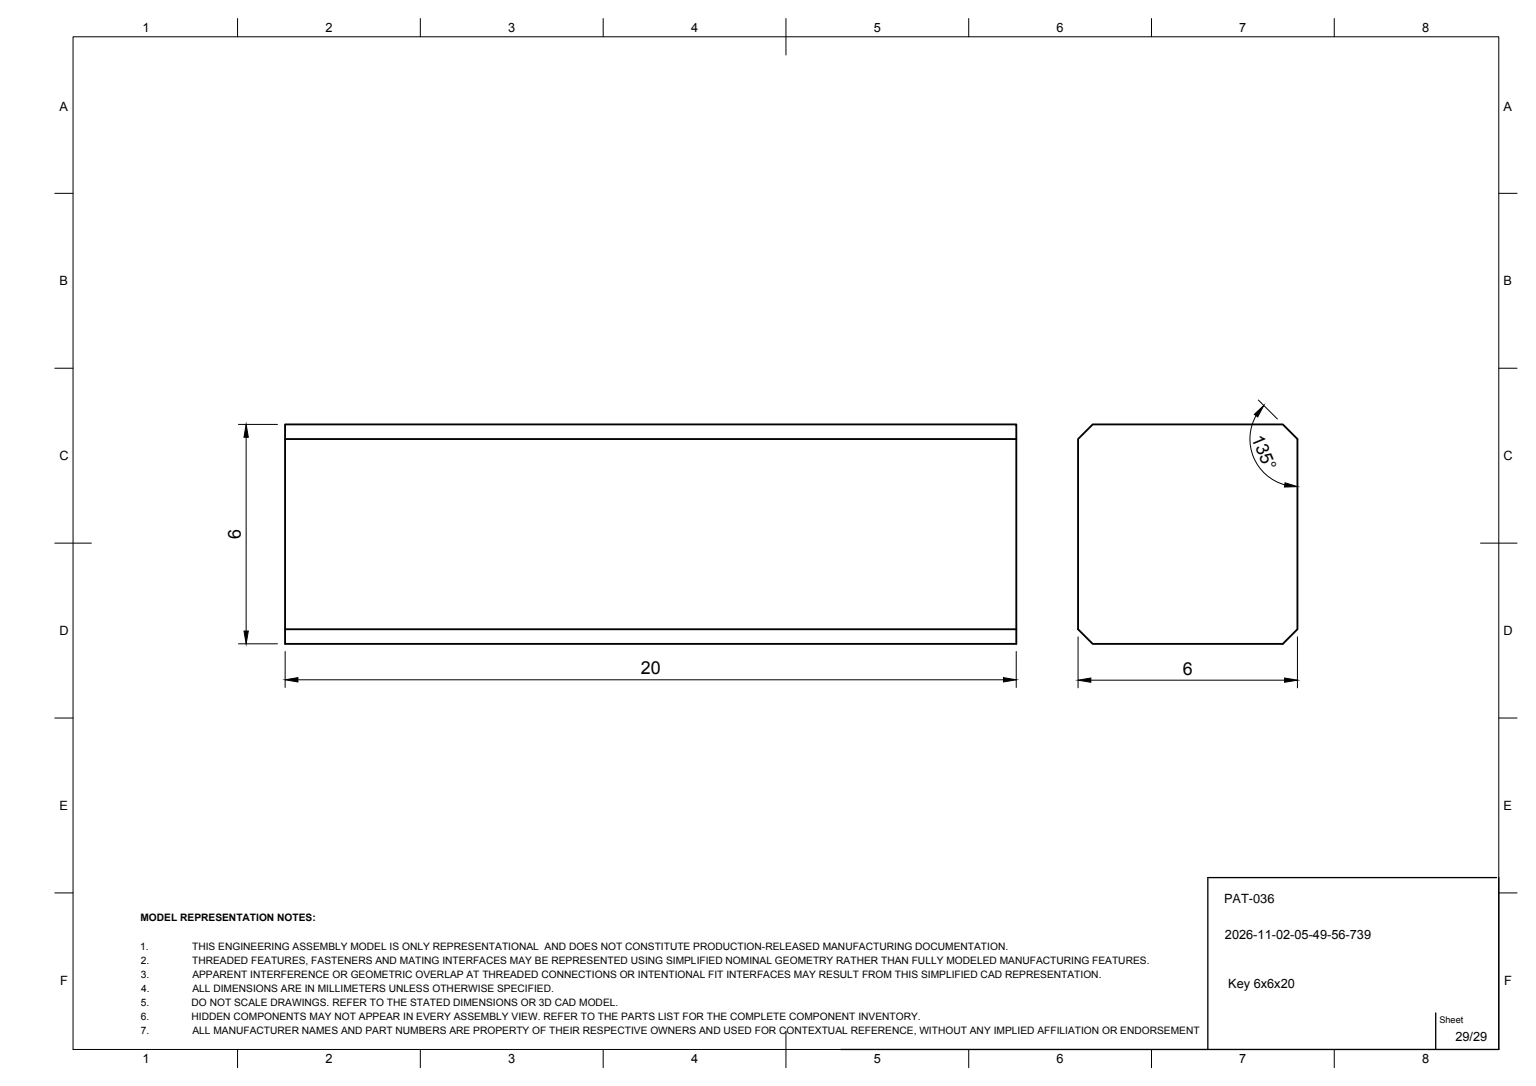
ISO-10303-21;
HEADER;
/* Generated by software containing ST-Developer
 * from STEP Tools, Inc. (www.steptools.com) 
 */

FILE_DESCRIPTION(
/* description */ ('Flange-mounted spindle'),
/* implementation_level */ '2;1');

FILE_NAME(
/* name */ 'Key 6x6x20.step',
/* time_stamp */ '2026-10-27T10:49:51-07:00',
/* author */ (''),
/* organization */ (''),
/* preprocessor_version */ 'ST-DEVELOPER v20.2',
/* originating_system */ 'Autodesk Translation Framework v15.17.0.0',
/* authorisation */ '');

FILE_SCHEMA (('AUTOMOTIVE_DESIGN { 1 0 10303 214 3 1 1 }'));
ENDSEC;

DATA;
#10=MECHANICAL_DESIGN_GEOMETRIC_PRESENTATION_REPRESENTATION('',(#363),#11764);
#308=SHAPE_REPRESENTATION_RELATIONSHIP('SRR','None',#11906,#335);
#335=ADVANCED_BREP_SHAPE_REPRESENTATION('',(#388),#11761);
#363=STYLED_ITEM('',(#12099),#388);
#388=MANIFOLD_SOLID_BREP('Body1',#6158);
#654=PLANE('',#7128);
#655=PLANE('',#7129);
#656=PLANE('',#7130);
#657=PLANE('',#7131);
#658=PLANE('',#7132);
#659=PLANE('',#7133);
#660=PLANE('',#7134);
#661=PLANE('',#7135);
#662=PLANE('',#7136);
#663=PLANE('',#7137);
#994=FACE_OUTER_BOUND('',#1450,.T.);
#995=FACE_OUTER_BOUND('',#1451,.T.);
#996=FACE_OUTER_BOUND('',#1452,.T.);
#997=FACE_OUTER_BOUND('',#1453,.T.);
#998=FACE_OUTER_BOUND('',#1454,.T.);
#999=FACE_OUTER_BOUND('',#1455,.T.);
#1000=FACE_OUTER_BOUND('',#1456,.T.);
#1001=FACE_OUTER_BOUND('',#1457,.T.);
#1002=FACE_OUTER_BOUND('',#1458,.T.);
#1003=FACE_OUTER_BOUND('',#1459,.T.);
#1450=EDGE_LOOP('',(#5515,#5516,#5517,#5518,#5519,#5520,#5521,#5522));
#1451=EDGE_LOOP('',(#5523,#5524,#5525,#5526));
#1452=EDGE_LOOP('',(#5527,#5528,#5529,#5530));
#1453=EDGE_LOOP('',(#5531,#5532,#5533,#5534));
#1454=EDGE_LOOP('',(#5535,#5536,#5537,#5538));
#1455=EDGE_LOOP('',(#5539,#5540,#5541,#5542,#5543,#5544,#5545,#5546));
#1456=EDGE_LOOP('',(#5547,#5548,#5549,#5550));
#1457=EDGE_LOOP('',(#5551,#5552,#5553,#5554));
#1458=EDGE_LOOP('',(#5555,#5556,#5557,#5558));
#1459=EDGE_LOOP('',(#5559,#5560,#5561,#5562));
#1866=LINE('',#11517,#2288);
#1867=LINE('',#11519,#2289);
#1868=LINE('',#11521,#2290);
#1869=LINE('',#11523,#2291);
#1870=LINE('',#11525,#2292);
#1871=LINE('',#11527,#2293);
#1872=LINE('',#11529,#2294);
#1873=LINE('',#11530,#2295);
#1874=LINE('',#11533,#2296);
#1875=LINE('',#11535,#2297);
#1876=LINE('',#11536,#2298);
#1877=LINE('',#11539,#2299);
#1878=LINE('',#11540,#2300);
#1879=LINE('',#11543,#2301);
#1880=LINE('',#11544,#2302);
#1881=LINE('',#11547,#2303);
#1882=LINE('',#11548,#2304);
#1883=LINE('',#11552,#2305);
#1884=LINE('',#11553,#2306);
#1885=LINE('',#11555,#2307);
#1886=LINE('',#11556,#2308);
#1887=LINE('',#11558,#2309);
#1888=LINE('',#11560,#2310);
#1889=LINE('',#11562,#2311);
#2288=VECTOR('',#8935,1.);
#2289=VECTOR('',#8936,1.);
#2290=VECTOR('',#8937,1.);
#2291=VECTOR('',#8938,1.);
#2292=VECTOR('',#8939,1.);
#2293=VECTOR('',#8940,1.);
#2294=VECTOR('',#8941,1.);
#2295=VECTOR('',#8942,1.);
#2296=VECTOR('',#8945,1.);
#2297=VECTOR('',#8946,1.);
#2298=VECTOR('',#8947,1.);
#2299=VECTOR('',#8950,1.);
#2300=VECTOR('',#8951,1.);
#2301=VECTOR('',#8954,1.);
#2302=VECTOR('',#8955,1.);
#2303=VECTOR('',#8958,1.);
#2304=VECTOR('',#8959,1.);
#2305=VECTOR('',#8962,1.);
#2306=VECTOR('',#8963,1.);
#2307=VECTOR('',#8964,1.);
#2308=VECTOR('',#8965,1.);
#2309=VECTOR('',#8968,1.);
#2310=VECTOR('',#8971,1.);
#2311=VECTOR('',#8974,1.);
#3159=VERTEX_POINT('',#11515);
#3160=VERTEX_POINT('',#11516);
#3161=VERTEX_POINT('',#11518);
#3162=VERTEX_POINT('',#11520);
#3163=VERTEX_POINT('',#11522);
#3164=VERTEX_POINT('',#11524);
#3165=VERTEX_POINT('',#11526);
#3166=VERTEX_POINT('',#11528);
#3167=VERTEX_POINT('',#11532);
#3168=VERTEX_POINT('',#11534);
#3169=VERTEX_POINT('',#11538);
#3170=VERTEX_POINT('',#11542);
#3171=VERTEX_POINT('',#11546);
#3172=VERTEX_POINT('',#11550);
#3173=VERTEX_POINT('',#11551);
#3174=VERTEX_POINT('',#11554);
#3950=EDGE_CURVE('',#3159,#3160,#1866,.T.);
#3951=EDGE_CURVE('',#3161,#3159,#1867,.T.);
#3952=EDGE_CURVE('',#3162,#3161,#1868,.T.);
#3953=EDGE_CURVE('',#3163,#3162,#1869,.T.);
#3954=EDGE_CURVE('',#3164,#3163,#1870,.T.);
#3955=EDGE_CURVE('',#3165,#3164,#1871,.T.);
#3956=EDGE_CURVE('',#3166,#3165,#1872,.T.);
#3957=EDGE_CURVE('',#3160,#3166,#1873,.T.);
#3958=EDGE_CURVE('',#3163,#3167,#1874,.T.);
#3959=EDGE_CURVE('',#3167,#3168,#1875,.T.);
#3960=EDGE_CURVE('',#3168,#3164,#1876,.T.);
#3961=EDGE_CURVE('',#3169,#3162,#1877,.T.);
#3962=EDGE_CURVE('',#3169,#3167,#1878,.T.);
#3963=EDGE_CURVE('',#3161,#3170,#1879,.T.);
#3964=EDGE_CURVE('',#3170,#3169,#1880,.T.);
#3965=EDGE_CURVE('',#3171,#3159,#1881,.T.);
#3966=EDGE_CURVE('',#3171,#3170,#1882,.T.);
#3967=EDGE_CURVE('',#3172,#3173,#1883,.T.);
#3968=EDGE_CURVE('',#3168,#3172,#1884,.T.);
#3969=EDGE_CURVE('',#3174,#3171,#1885,.T.);
#3970=EDGE_CURVE('',#3173,#3174,#1886,.T.);
#3971=EDGE_CURVE('',#3165,#3172,#1887,.T.);
#3972=EDGE_CURVE('',#3160,#3174,#1888,.T.);
#3973=EDGE_CURVE('',#3173,#3166,#1889,.T.);
#5515=ORIENTED_EDGE('',*,*,#3950,.F.);
#5516=ORIENTED_EDGE('',*,*,#3951,.F.);
#5517=ORIENTED_EDGE('',*,*,#3952,.F.);
#5518=ORIENTED_EDGE('',*,*,#3953,.F.);
#5519=ORIENTED_EDGE('',*,*,#3954,.F.);
#5520=ORIENTED_EDGE('',*,*,#3955,.F.);
#5521=ORIENTED_EDGE('',*,*,#3956,.F.);
#5522=ORIENTED_EDGE('',*,*,#3957,.F.);
#5523=ORIENTED_EDGE('',*,*,#3954,.T.);
#5524=ORIENTED_EDGE('',*,*,#3958,.T.);
#5525=ORIENTED_EDGE('',*,*,#3959,.T.);
#5526=ORIENTED_EDGE('',*,*,#3960,.T.);
#5527=ORIENTED_EDGE('',*,*,#3953,.T.);
#5528=ORIENTED_EDGE('',*,*,#3961,.F.);
#5529=ORIENTED_EDGE('',*,*,#3962,.T.);
#5530=ORIENTED_EDGE('',*,*,#3958,.F.);
#5531=ORIENTED_EDGE('',*,*,#3952,.T.);
#5532=ORIENTED_EDGE('',*,*,#3963,.T.);
#5533=ORIENTED_EDGE('',*,*,#3964,.T.);
#5534=ORIENTED_EDGE('',*,*,#3961,.T.);
#5535=ORIENTED_EDGE('',*,*,#3951,.T.);
#5536=ORIENTED_EDGE('',*,*,#3965,.F.);
#5537=ORIENTED_EDGE('',*,*,#3966,.T.);
#5538=ORIENTED_EDGE('',*,*,#3963,.F.);
#5539=ORIENTED_EDGE('',*,*,#3967,.F.);
#5540=ORIENTED_EDGE('',*,*,#3968,.F.);
#5541=ORIENTED_EDGE('',*,*,#3959,.F.);
#5542=ORIENTED_EDGE('',*,*,#3962,.F.);
#5543=ORIENTED_EDGE('',*,*,#3964,.F.);
#5544=ORIENTED_EDGE('',*,*,#3966,.F.);
#5545=ORIENTED_EDGE('',*,*,#3969,.F.);
#5546=ORIENTED_EDGE('',*,*,#3970,.F.);
#5547=ORIENTED_EDGE('',*,*,#3955,.T.);
#5548=ORIENTED_EDGE('',*,*,#3960,.F.);
#5549=ORIENTED_EDGE('',*,*,#3968,.T.);
#5550=ORIENTED_EDGE('',*,*,#3971,.F.);
#5551=ORIENTED_EDGE('',*,*,#3950,.T.);
#5552=ORIENTED_EDGE('',*,*,#3972,.T.);
#5553=ORIENTED_EDGE('',*,*,#3969,.T.);
#5554=ORIENTED_EDGE('',*,*,#3965,.T.);
#5555=ORIENTED_EDGE('',*,*,#3956,.T.);
#5556=ORIENTED_EDGE('',*,*,#3971,.T.);
#5557=ORIENTED_EDGE('',*,*,#3967,.T.);
#5558=ORIENTED_EDGE('',*,*,#3973,.T.);
#5559=ORIENTED_EDGE('',*,*,#3957,.T.);
#5560=ORIENTED_EDGE('',*,*,#3973,.F.);
#5561=ORIENTED_EDGE('',*,*,#3970,.T.);
#5562=ORIENTED_EDGE('',*,*,#3972,.F.);
#6105=ADVANCED_FACE('',(#994),#654,.F.);
#6106=ADVANCED_FACE('',(#995),#655,.T.);
#6107=ADVANCED_FACE('',(#996),#656,.T.);
#6108=ADVANCED_FACE('',(#997),#657,.T.);
#6109=ADVANCED_FACE('',(#998),#658,.T.);
#6110=ADVANCED_FACE('',(#999),#659,.T.);
#6111=ADVANCED_FACE('',(#1000),#660,.F.);
#6112=ADVANCED_FACE('',(#1001),#661,.T.);
#6113=ADVANCED_FACE('',(#1002),#662,.T.);
#6114=ADVANCED_FACE('',(#1003),#663,.T.);
#6158=CLOSED_SHELL('',(#6105,#6106,#6107,#6108,#6109,#6110,#6111,#6112,
#6113,#6114));
#7127=AXIS2_PLACEMENT_3D('',#11513,#8931,#8932);
#7128=AXIS2_PLACEMENT_3D('',#11514,#8933,#8934);
#7129=AXIS2_PLACEMENT_3D('',#11531,#8943,#8944);
#7130=AXIS2_PLACEMENT_3D('',#11537,#8948,#8949);
#7131=AXIS2_PLACEMENT_3D('',#11541,#8952,#8953);
#7132=AXIS2_PLACEMENT_3D('',#11545,#8956,#8957);
#7133=AXIS2_PLACEMENT_3D('',#11549,#8960,#8961);
#7134=AXIS2_PLACEMENT_3D('',#11557,#8966,#8967);
#7135=AXIS2_PLACEMENT_3D('',#11559,#8969,#8970);
#7136=AXIS2_PLACEMENT_3D('',#11561,#8972,#8973);
#7137=AXIS2_PLACEMENT_3D('',#11563,#8975,#8976);
#8931=DIRECTION('axis',(0.,0.,1.));
#8932=DIRECTION('refdir',(1.,0.,0.));
#8933=DIRECTION('center_axis',(1.,0.,0.));
#8934=DIRECTION('ref_axis',(0.,0.,-1.));
#8935=DIRECTION('',(0.,-0.707106781186547,-0.707106781186548));
#8936=DIRECTION('',(0.,-1.,0.));
#8937=DIRECTION('',(0.,-0.707106781186547,0.707106781186548));
#8938=DIRECTION('',(0.,0.,1.));
#8939=DIRECTION('',(0.,0.707106781186547,0.707106781186548));
#8940=DIRECTION('',(0.,1.,0.));
#8941=DIRECTION('',(0.,0.707106781186547,-0.707106781186548));
#8942=DIRECTION('',(0.,0.,-1.));
#8943=DIRECTION('center_axis',(0.,0.707106781186548,-0.707106781186547));
#8944=DIRECTION('ref_axis',(-1.,0.,0.));
#8945=DIRECTION('',(1.,0.,0.));
#8946=DIRECTION('',(0.,-0.707106781186547,-0.707106781186548));
#8947=DIRECTION('',(-1.,0.,0.));
#8948=DIRECTION('center_axis',(0.,1.,0.));
#8949=DIRECTION('ref_axis',(-1.,0.,0.));
#8950=DIRECTION('',(-1.,0.,0.));
#8951=DIRECTION('',(0.,0.,-1.));
#8952=DIRECTION('center_axis',(0.,0.707106781186548,0.707106781186547));
#8953=DIRECTION('ref_axis',(1.,0.,0.));
#8954=DIRECTION('',(1.,0.,0.));
#8955=DIRECTION('',(0.,0.707106781186547,-0.707106781186548));
#8956=DIRECTION('center_axis',(0.,0.,1.));
#8957=DIRECTION('ref_axis',(1.,0.,0.));
#8958=DIRECTION('',(-1.,0.,0.));
#8959=DIRECTION('',(0.,1.,0.));
#8960=DIRECTION('center_axis',(1.,0.,0.));
#8961=DIRECTION('ref_axis',(0.,0.,-1.));
#8962=DIRECTION('',(0.,-0.707106781186547,0.707106781186548));
#8963=DIRECTION('',(0.,-1.,0.));
#8964=DIRECTION('',(0.,0.707106781186547,0.707106781186548));
#8965=DIRECTION('',(0.,0.,1.));
#8966=DIRECTION('center_axis',(0.,0.,1.));
#8967=DIRECTION('ref_axis',(1.,0.,0.));
#8968=DIRECTION('',(1.,0.,0.));
#8969=DIRECTION('center_axis',(0.,-0.707106781186548,0.707106781186547));
#8970=DIRECTION('ref_axis',(1.,0.,0.));
#8971=DIRECTION('',(1.,0.,0.));
#8972=DIRECTION('center_axis',(0.,-0.707106781186548,-0.707106781186547));
#8973=DIRECTION('ref_axis',(-1.,0.,0.));
#8974=DIRECTION('',(-1.,0.,0.));
#8975=DIRECTION('center_axis',(0.,-1.,0.));
#8976=DIRECTION('ref_axis',(1.,0.,0.));
#11513=CARTESIAN_POINT('',(0.,0.,0.));
#11514=CARTESIAN_POINT('Origin',(-1.,0.,0.35));
#11515=CARTESIAN_POINT('',(-1.,-0.26,0.6));
#11516=CARTESIAN_POINT('',(-1.,-0.3,0.56));
#11517=CARTESIAN_POINT('',(-1.,-0.2675,0.5925));
#11518=CARTESIAN_POINT('',(-1.,0.26,0.6));
#11519=CARTESIAN_POINT('',(-1.,0.,0.6));
#11520=CARTESIAN_POINT('',(-1.,0.3,0.56));
#11521=CARTESIAN_POINT('',(-1.,0.2675,0.5925));
#11522=CARTESIAN_POINT('',(-1.,0.3,0.04));
#11523=CARTESIAN_POINT('',(-1.,0.3,0.175));
#11524=CARTESIAN_POINT('',(-1.,0.26,0.));
#11525=CARTESIAN_POINT('',(-1.,0.2925,0.0325));
#11526=CARTESIAN_POINT('',(-1.,-0.26,0.));
#11527=CARTESIAN_POINT('',(-1.,0.,0.));
#11528=CARTESIAN_POINT('',(-1.,-0.3,0.04));
#11529=CARTESIAN_POINT('',(-1.,-0.2925,0.0325));
#11530=CARTESIAN_POINT('',(-1.,-0.3,0.175));
#11531=CARTESIAN_POINT('Origin',(0.75,0.28,0.02));
#11532=CARTESIAN_POINT('',(1.,0.3,0.04));
#11533=CARTESIAN_POINT('',(0.75,0.3,0.04));
#11534=CARTESIAN_POINT('',(1.,0.26,0.));
#11535=CARTESIAN_POINT('',(1.,0.2925,0.0325));
#11536=CARTESIAN_POINT('',(0.75,0.26,0.));
#11537=CARTESIAN_POINT('Origin',(1.5,0.3,0.));
#11538=CARTESIAN_POINT('',(1.,0.3,0.56));
#11539=CARTESIAN_POINT('',(0.75,0.3,0.56));
#11540=CARTESIAN_POINT('',(1.,0.3,0.175));
#11541=CARTESIAN_POINT('Origin',(0.75,0.28,0.58));
#11542=CARTESIAN_POINT('',(1.,0.26,0.6));
#11543=CARTESIAN_POINT('',(0.75,0.26,0.6));
#11544=CARTESIAN_POINT('',(1.,0.2675,0.5925));
#11545=CARTESIAN_POINT('Origin',(0.,0.,0.6));
#11546=CARTESIAN_POINT('',(1.,-0.26,0.6));
#11547=CARTESIAN_POINT('',(-0.75,-0.26,0.6));
#11548=CARTESIAN_POINT('',(1.,0.,0.6));
#11549=CARTESIAN_POINT('Origin',(1.,0.,0.35));
#11550=CARTESIAN_POINT('',(1.,-0.26,0.));
#11551=CARTESIAN_POINT('',(1.,-0.3,0.04));
#11552=CARTESIAN_POINT('',(1.,-0.2925,0.0325));
#11553=CARTESIAN_POINT('',(1.,0.,0.));
#11554=CARTESIAN_POINT('',(1.,-0.3,0.56));
#11555=CARTESIAN_POINT('',(1.,-0.2675,0.5925));
#11556=CARTESIAN_POINT('',(1.,-0.3,0.175));
#11557=CARTESIAN_POINT('Origin',(0.,0.,0.));
#11558=CARTESIAN_POINT('',(-0.75,-0.26,0.));
#11559=CARTESIAN_POINT('Origin',(-0.75,-0.28,0.58));
#11560=CARTESIAN_POINT('',(-0.75,-0.3,0.56));
#11561=CARTESIAN_POINT('Origin',(-0.75,-0.28,0.02));
#11562=CARTESIAN_POINT('',(-0.75,-0.3,0.04));
#11563=CARTESIAN_POINT('Origin',(-1.5,-0.3,0.));
#11729=UNCERTAINTY_MEASURE_WITH_UNIT(LENGTH_MEASURE(0.001),#11765,
'DISTANCE_ACCURACY_VALUE',
'Maximum model space distance between geometric entities at asserted c
onnectivities');
#11732=UNCERTAINTY_MEASURE_WITH_UNIT(LENGTH_MEASURE(0.001),#11765,
'DISTANCE_ACCURACY_VALUE',
'Maximum model space distance between geometric entities at asserted c
onnectivities');
#11761=(
GEOMETRIC_REPRESENTATION_CONTEXT(3)
GLOBAL_UNCERTAINTY_ASSIGNED_CONTEXT((#11729))
GLOBAL_UNIT_ASSIGNED_CONTEXT((#11765,#11767,#11768))
REPRESENTATION_CONTEXT('','3D')
);
#11764=(
GEOMETRIC_REPRESENTATION_CONTEXT(3)
GLOBAL_UNCERTAINTY_ASSIGNED_CONTEXT((#11732))
GLOBAL_UNIT_ASSIGNED_CONTEXT((#11765,#11767,#11768))
REPRESENTATION_CONTEXT('','3D')
);
#11765=(
LENGTH_UNIT()
NAMED_UNIT(*)
SI_UNIT(.CENTI.,.METRE.)
);
#11767=(
NAMED_UNIT(*)
PLANE_ANGLE_UNIT()
SI_UNIT($,.RADIAN.)
);
#11768=(
NAMED_UNIT(*)
SI_UNIT($,.STERADIAN.)
SOLID_ANGLE_UNIT()
);
#11797=SHAPE_DEFINITION_REPRESENTATION(#11830,#11906);
#11830=PRODUCT_DEFINITION_SHAPE('',$,#11938);
#11906=SHAPE_REPRESENTATION('',(#7127),#11761);
#11909=PRODUCT_DEFINITION_CONTEXT('part definition',#12004,'design');
#11938=PRODUCT_DEFINITION('Key 6x6x20','Key 6x6x20',#11969,#11909);
#11969=PRODUCT_DEFINITION_FORMATION('',$,#12034);
#12004=APPLICATION_CONTEXT(
'Core Data for Automotive Mechanical Design Process');
#12005=PRODUCT_CONTEXT('part definition',#12004,'mechanical');
#12034=PRODUCT('Key 6x6x20','Key 6x6x20','Key 6x6x20',(#12005));
#12093=COLOUR_RGB('Grey',0.48,0.52,0.57);
#12094=FILL_AREA_STYLE_COLOUR('',#12093);
#12095=FILL_AREA_STYLE('',(#12094));
#12096=SURFACE_STYLE_FILL_AREA(#12095);
#12097=SURFACE_SIDE_STYLE('',(#12096));
#12098=SURFACE_STYLE_USAGE(.BOTH.,#12097);
#12099=PRESENTATION_STYLE_ASSIGNMENT((#12098));
ENDSEC;
END-ISO-10303-21;
